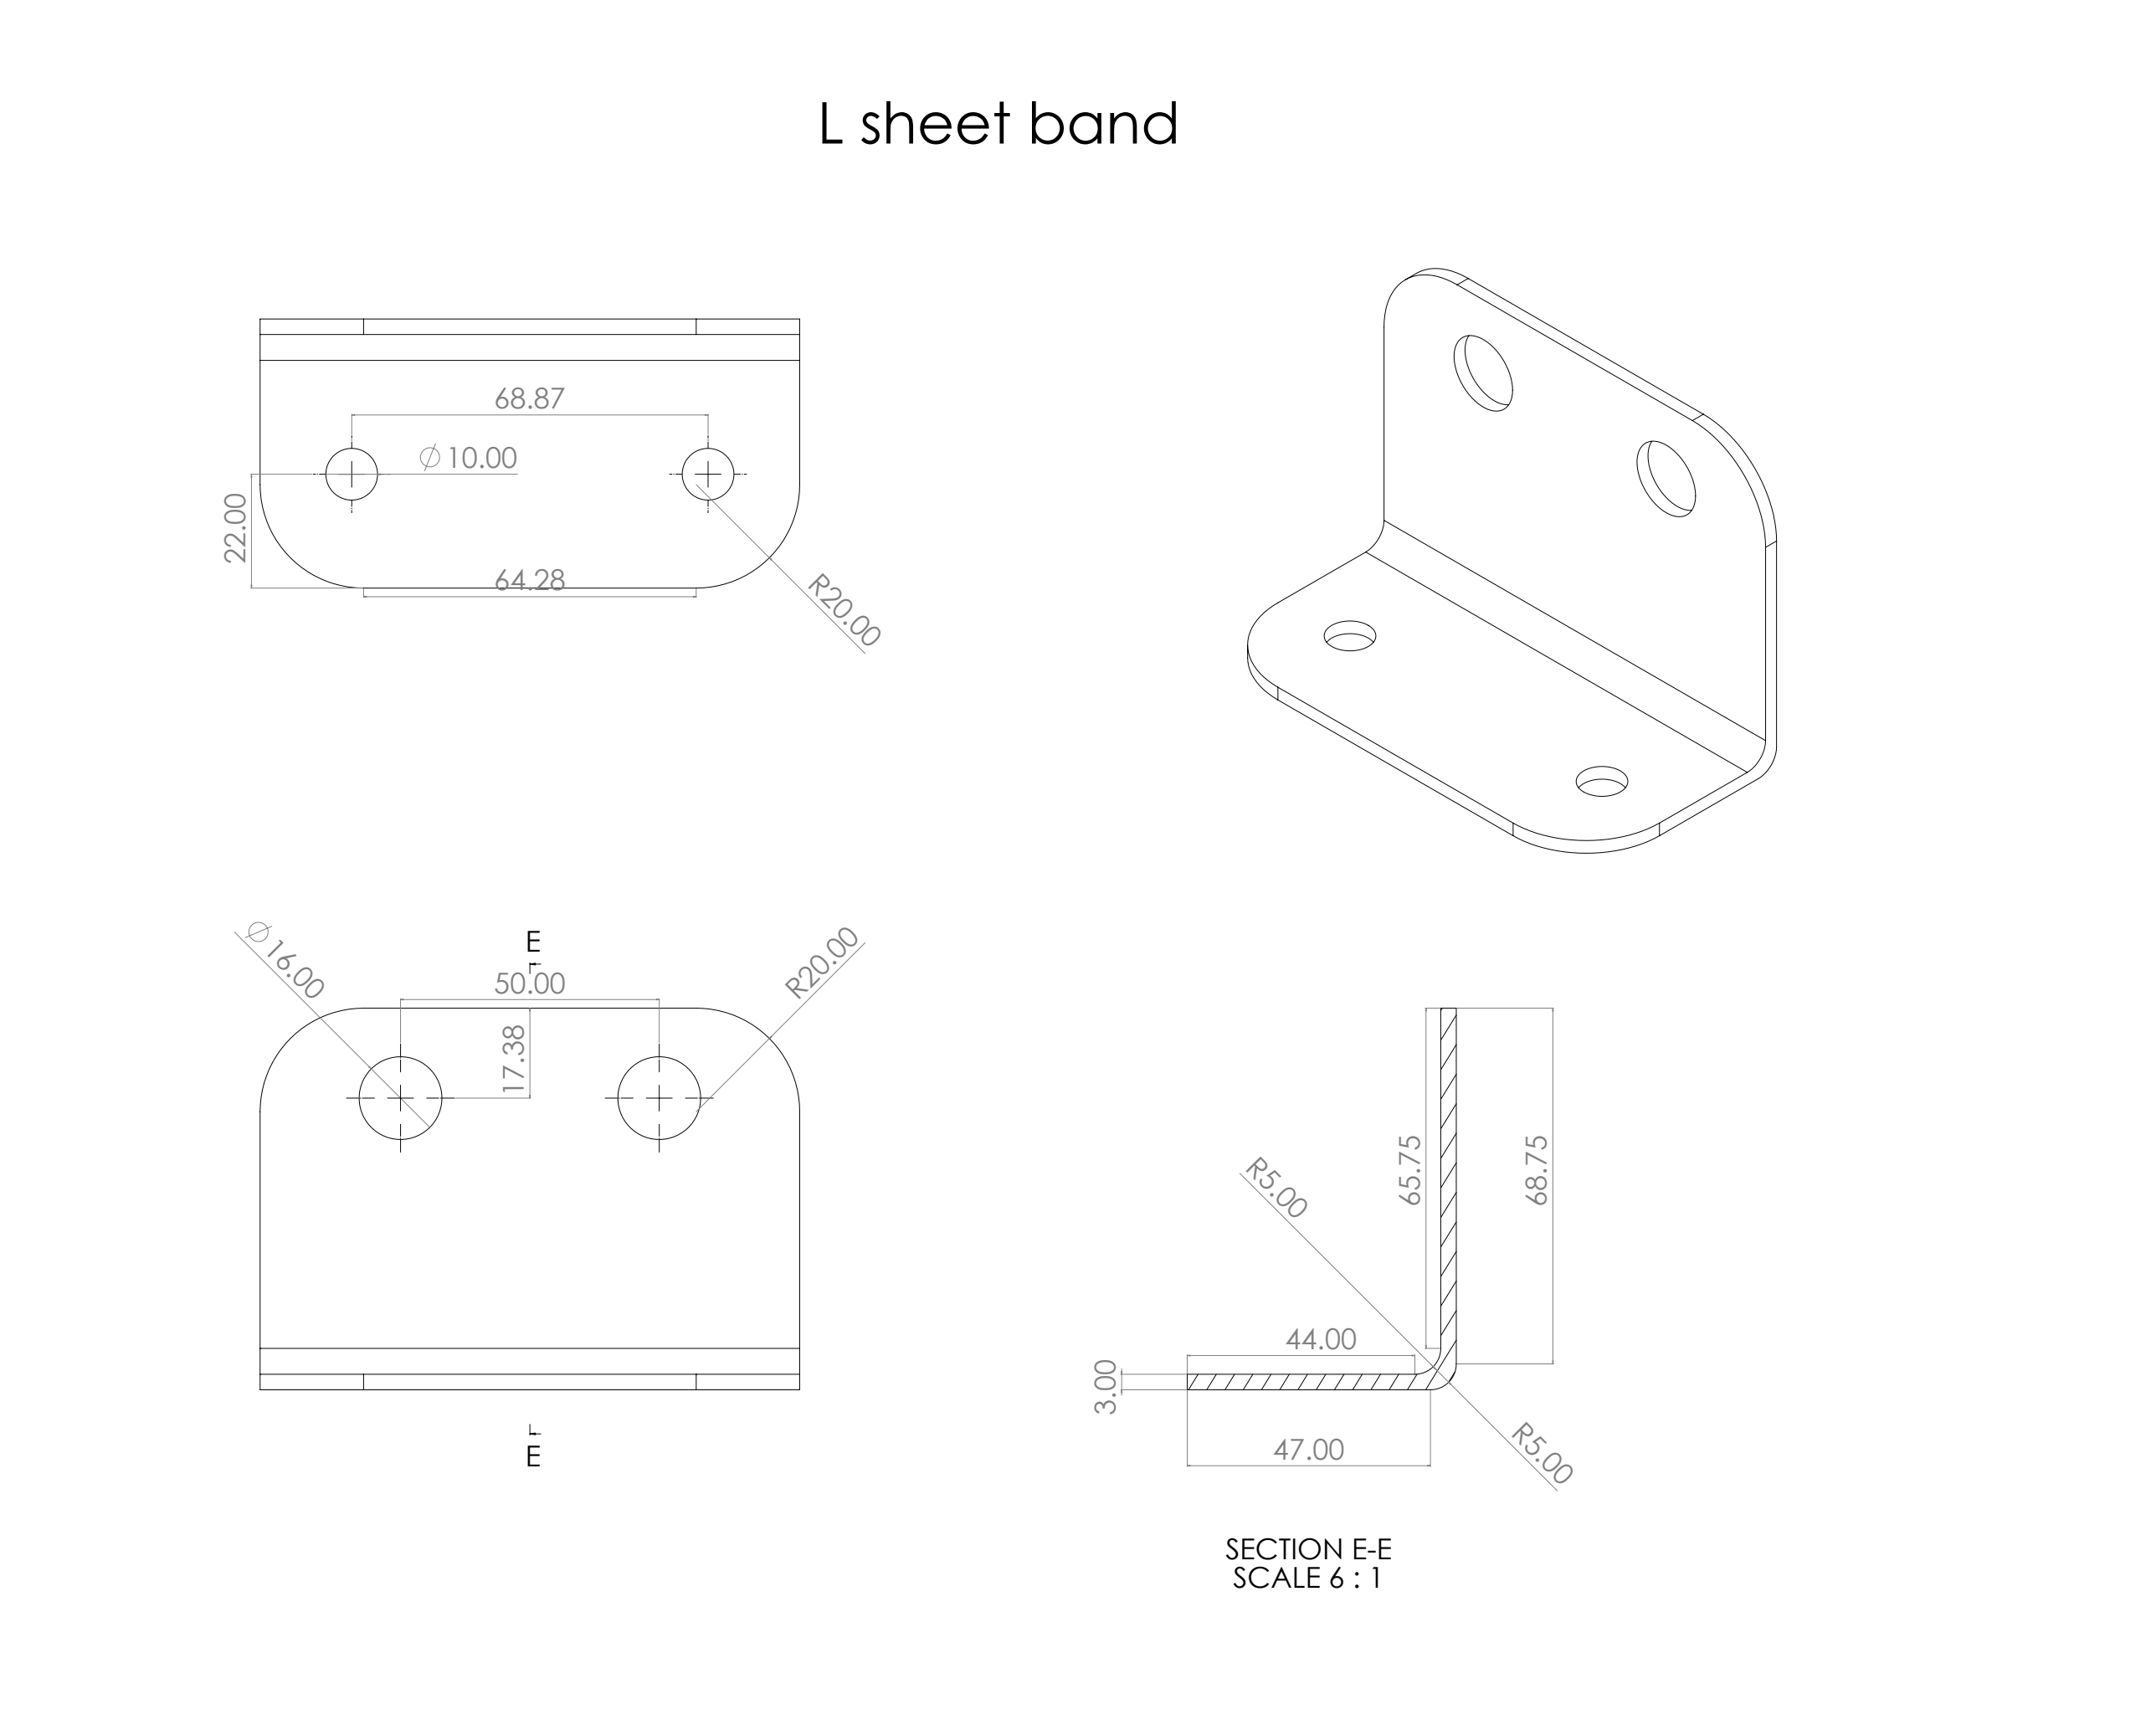
ISO-10303-21;
HEADER;
FILE_DESCRIPTION (('STEP AP214'),
    '1' );
FILE_NAME ('L sheet band.step',
    '2026-10-25T20:52:49',
    ( '' ),
    ( '' ),
    'SwSTEP 2.0',
    'SolidWorks 2025',
    '' );
FILE_SCHEMA (( 'AUTOMOTIVE_DESIGN' ));
ENDSEC;

DATA;
#211=CIRCLE ( 'NONE', #62253, 4.999999999999997335 ) ;
#499=ORIENTED_EDGE ( 'NONE', *, *, #5733, .T. ) ;
#503=CARTESIAN_POINT ( 'NONE',  ( -74.94434090351494149, -285.8906705383787994, 27.50000000000000000 ) ) ;
#530=CIRCLE ( 'NONE', #89712, 8.000000000000000000 ) ;
#590=VECTOR ( 'NONE', #42774, 1000.000000000000000 ) ;
#594=DIRECTION ( 'NONE',  ( -0.000000000000000000, 0.000000000000000000, -1.000000000000000000 ) ) ;
#669=ORIENTED_EDGE ( 'NONE', *, *, #93158, .F. ) ;
#679=EDGE_CURVE ( 'NONE', #83322, #83798, #47998, .T. ) ;
#791=EDGE_CURVE ( 'NONE', #63802, #44165, #5422, .T. ) ;
#865=ADVANCED_FACE ( 'NONE', ( #48951 ), #63665, .F. ) ;
#929=APPLICATION_CONTEXT ( 'automotive_design' ) ;
#1240=EDGE_CURVE ( 'NONE', #8882, #83322, #52548, .T. ) ;
#1428=ORIENTED_EDGE ( 'NONE', *, *, #14429, .F. ) ;
#1517=EDGE_LOOP ( 'NONE', ( #90741, #8726, #54853, #21935 ) ) ;
#1578=ORIENTED_EDGE ( 'NONE', *, *, #52624, .F. ) ;
#1600=CARTESIAN_POINT ( 'NONE',  ( 11.63197158325052172, -331.8906705383788562, 57.50000000000000000 ) ) ;
#1855=LINE ( 'NONE', #38761, #18792 ) ;
#1953=CIRCLE ( 'NONE', #71531, 5.000000000000000888 ) ;
#2043=AXIS2_PLACEMENT_3D ( 'NONE', #53323, #2683, #31562 ) ;
#2173=CIRCLE ( 'NONE', #35437, 20.00000000000000355 ) ;
#2187=VERTEX_POINT ( 'NONE', #4695 ) ;
#2252=( GEOMETRIC_REPRESENTATION_CONTEXT ( 3 ) GLOBAL_UNCERTAINTY_ASSIGNED_CONTEXT ( ( #85447 ) ) GLOBAL_UNIT_ASSIGNED_CONTEXT ( ( #20907, #28483, #57377 ) ) REPRESENTATION_CONTEXT ( 'NONE', 'WORKASPACE' ) );
#2451=VECTOR ( 'NONE', #84118, 1000.000000000000000 ) ;
#2470=CYLINDRICAL_SURFACE ( 'NONE', #63999, 5.000000000000004441 ) ;
#2536=ORIENTED_EDGE ( 'NONE', *, *, #16849, .T. ) ;
#2683=DIRECTION ( 'NONE',  ( -0.000000000000000000, 1.000000000000000000, -0.000000000000000000 ) ) ;
#2731=CARTESIAN_POINT ( 'NONE',  ( 29.33919985515026596, -285.8906705383787994, 25.50000000000000000 ) ) ;
#2748=LINE ( 'NONE', #18829, #53687 ) ;
#2764=ORIENTED_EDGE ( 'NONE', *, *, #65408, .F. ) ;
#3216=EDGE_CURVE ( 'NONE', #6956, #36970, #44399, .T. ) ;
#3291=FACE_BOUND ( 'NONE', #79678, .T. ) ;
#3472=EDGE_CURVE ( 'NONE', #2187, #79053, #42928, .T. ) ;
#3535=VECTOR ( 'NONE', #44027, 1000.000000000000000 ) ;
#3654=AXIS2_PLACEMENT_3D ( 'NONE', #5607, #71407, #86506 ) ;
#4161=DIRECTION ( 'NONE',  ( 0.000000000000000000, 0.000000000000000000, 1.000000000000000000 ) ) ;
#4211=CARTESIAN_POINT ( 'NONE',  ( 9.339199855150265961, -212.1443419142231051, 25.50000000000000000 ) ) ;
#4278=CYLINDRICAL_SURFACE ( 'NONE', #44327, 20.00000000000000355 ) ;
#4618=DIRECTION ( 'NONE',  ( -1.000000000000000000, 0.000000000000000000, 0.000000000000000000 ) ) ;
#4695=CARTESIAN_POINT ( 'NONE',  ( -57.23711263161519724, -282.8906705383787994, 47.50000000000000000 ) ) ;
#4733=ORIENTED_EDGE ( 'NONE', *, *, #61391, .F. ) ;
#4911=EDGE_CURVE ( 'NONE', #16098, #8882, #2173, .T. ) ;
#5333=ORIENTED_EDGE ( 'NONE', *, *, #71135, .T. ) ;
#5370=CARTESIAN_POINT ( 'NONE',  ( -74.94434090351494149, -232.1443419142230766, 25.50000000000000000 ) ) ;
#5378=CARTESIAN_POINT ( 'NONE',  ( -47.80257052418233599, -229.5268262511776527, 25.50000000000000000 ) ) ;
#5422=LINE ( 'NONE', #41357, #59082 ) ;
#5562=VERTEX_POINT ( 'NONE', #28040 ) ;
#5575=ORIENTED_EDGE ( 'NONE', *, *, #29965, .T. ) ;
#5605=FACE_OUTER_BOUND ( 'NONE', #91771, .T. ) ;
#5607=CARTESIAN_POINT ( 'NONE',  ( 9.339199855150265961, 0.000000000000000000, 54.50000000000000711 ) ) ;
#5696=DIRECTION ( 'NONE',  ( 0.000000000000000000, 0.000000000000000000, -1.000000000000000000 ) ) ;
#5733=EDGE_CURVE ( 'NONE', #83883, #21738, #35116, .T. ) ;
#5768=ORIENTED_EDGE ( 'NONE', *, *, #15154, .F. ) ;
#5834=CARTESIAN_POINT ( 'NONE',  ( 9.339199855150265961, -232.1443419142230766, 25.50000000000000000 ) ) ;
#5880=DIRECTION ( 'NONE',  ( -0.000000000000000000, 1.000000000000000000, -0.000000000000000000 ) ) ;
#6157=CIRCLE ( 'NONE', #21289, 5.000000000000004441 ) ;
#6190=CYLINDRICAL_SURFACE ( 'NONE', #46878, 20.00000000000000355 ) ;
#6253=ORIENTED_EDGE ( 'NONE', *, *, #81207, .T. ) ;
#6304=DIRECTION ( 'NONE',  ( 1.000000000000000000, 0.000000000000000000, -0.000000000000000000 ) ) ;
#6314=EDGE_LOOP ( 'NONE', ( #19635, #51769, #6625, #41760 ) ) ;
#6319=EDGE_LOOP ( 'NONE', ( #54530, #85626, #35666, #19153 ) ) ;
#6408=CARTESIAN_POINT ( 'NONE',  ( 11.63197158325052172, -282.8906705383787994, 52.50000000000000711 ) ) ;
#6625=ORIENTED_EDGE ( 'NONE', *, *, #39536, .F. ) ;
#6628=AXIS2_PLACEMENT_3D ( 'NONE', #41896, #20617, #63257 ) ;
#6848=EDGE_LOOP ( 'NONE', ( #78571, #68659, #63310, #44201 ) ) ;
#6956=VERTEX_POINT ( 'NONE', #81914 ) ;
#7018=CARTESIAN_POINT ( 'NONE',  ( 9.339199855150262408, -285.8906705383787994, 74.50000000000001421 ) ) ;
#7577=DIRECTION ( 'NONE',  ( 0.000000000000000000, 0.000000000000000000, 1.000000000000000000 ) ) ;
#7662=EDGE_CURVE ( 'NONE', #46169, #75426, #44596, .T. ) ;
#7944=ORIENTED_EDGE ( 'NONE', *, *, #679, .T. ) ;
#8045=AXIS2_PLACEMENT_3D ( 'NONE', #26662, #19096, #40362 ) ;
#8145=FACE_OUTER_BOUND ( 'NONE', #43480, .T. ) ;
#8181=AXIS2_PLACEMENT_3D ( 'NONE', #46720, #18327, #89815 ) ;
#8225=VERTEX_POINT ( 'NONE', #32625 ) ;
#8251=VECTOR ( 'NONE', #27083, 1000.000000000000000 ) ;
#8548=ORIENTED_EDGE ( 'NONE', *, *, #29467, .T. ) ;
#8578=DIRECTION ( 'NONE',  ( -0.000000000000000000, 1.000000000000000000, -0.000000000000000000 ) ) ;
#8726=ORIENTED_EDGE ( 'NONE', *, *, #56813, .T. ) ;
#8882=VERTEX_POINT ( 'NONE', #7018 ) ;
#9133=VERTEX_POINT ( 'NONE', #16318 ) ;
#9154=DIRECTION ( 'NONE',  ( -1.000000000000000000, 0.000000000000000000, 0.000000000000000000 ) ) ;
#9364=CIRCLE ( 'NONE', #22964, 20.00000000000000000 ) ;
#9380=ORIENTED_EDGE ( 'NONE', *, *, #53233, .F. ) ;
#9395=LINE ( 'NONE', #66263, #77580 ) ;
#9712=AXIS2_PLACEMENT_3D ( 'NONE', #80216, #9154, #87304 ) ;
#9773=CARTESIAN_POINT ( 'NONE',  ( -39.80257052418233599, -229.5268262511776527, 22.50000000000000000 ) ) ;
#9810=AXIS2_PLACEMENT_3D ( 'NONE', #43476, #35459, #57245 ) ;
#9965=ORIENTED_EDGE ( 'NONE', *, *, #36530, .F. ) ;
#9996=MECHANICAL_DESIGN_GEOMETRIC_PRESENTATION_REPRESENTATION('',(#22120),#64479);
#10069=ADVANCED_FACE ( 'NONE', ( #63173 ), #41332, .F. ) ;
#10083=ORIENTED_EDGE ( 'NONE', *, *, #3472, .F. ) ;
#10105=EDGE_CURVE ( 'NONE', #5562, #61290, #30617, .T. ) ;
#10228=DIRECTION ( 'NONE',  ( 1.000000000000000000, 0.000000000000000000, -0.000000000000000000 ) ) ;
#10503=ORIENTED_EDGE ( 'NONE', *, *, #50543, .T. ) ;
#10525=CARTESIAN_POINT ( 'NONE',  ( 9.339199855150265961, -285.8906705383787994, 54.50000000000000711 ) ) ;
#10708=DIRECTION ( 'NONE',  ( -0.000000000000000000, -1.000000000000000000, 0.000000000000000000 ) ) ;
#10810=CARTESIAN_POINT ( 'NONE',  ( 29.33919985515026596, -282.8906705383787994, 74.50000000000001421 ) ) ;
#10935=EDGE_CURVE ( 'NONE', #74457, #43263, #11136, .T. ) ;
#11136=CIRCLE ( 'NONE', #77668, 5.000000000000000888 ) ;
#11171=DIRECTION ( 'NONE',  ( -1.000000000000000000, -0.000000000000000000, 0.000000000000000000 ) ) ;
#11303=CIRCLE ( 'NONE', #85390, 8.000000000000000000 ) ;
#11310=UNCERTAINTY_MEASURE_WITH_UNIT (LENGTH_MEASURE( 1.000000000000000082E-05 ), #27421, 'distance_accuracy_value', 'NONE');
#11330=DIRECTION ( 'NONE',  ( 1.000000000000000000, 0.000000000000000000, 0.000000000000000000 ) ) ;
#11515=FACE_OUTER_BOUND ( 'NONE', #28357, .T. ) ;
#11619=DIRECTION ( 'NONE',  ( 0.000000000000000000, 0.000000000000000000, 1.000000000000000000 ) ) ;
#12027=AXIS2_PLACEMENT_3D ( 'NONE', #47486, #46093, #82550 ) ;
#12043=EDGE_LOOP ( 'NONE', ( #77514, #31253 ) ) ;
#12155=VECTOR ( 'NONE', #33086, 1000.000000000000000 ) ;
#12164=ORIENTED_EDGE ( 'NONE', *, *, #57750, .F. ) ;
#12388=EDGE_LOOP ( 'NONE', ( #84486, #669, #4733, #84122 ) ) ;
#12459=ORIENTED_EDGE ( 'NONE', *, *, #52360, .T. ) ;
#12648=ORIENTED_EDGE ( 'NONE', *, *, #28991, .T. ) ;
#12657=PRODUCT_DEFINITION_SHAPE ( 'NONE', 'NONE',  #79429 ) ;
#12775=ORIENTED_EDGE ( 'NONE', *, *, #36530, .T. ) ;
#13302=DIRECTION ( 'NONE',  ( 0.000000000000000000, 0.000000000000000000, -1.000000000000000000 ) ) ;
#13640=CARTESIAN_POINT ( 'NONE',  ( 29.33919985515026596, -285.8906705383787994, 25.50000000000000000 ) ) ;
#13872=AXIS2_PLACEMENT_3D ( 'NONE', #69873, #11171, #24921 ) ;
#14429=EDGE_CURVE ( 'NONE', #21926, #45777, #1855, .T. ) ;
#14585=CARTESIAN_POINT ( 'NONE',  ( 29.33919985515026596, -280.8906705383787994, 22.50000000000000000 ) ) ;
#14821=ORIENTED_EDGE ( 'NONE', *, *, #679, .F. ) ;
#14991=DIRECTION ( 'NONE',  ( -1.000000000000000000, 0.000000000000000000, 0.000000000000000000 ) ) ;
#15070=CIRCLE ( 'NONE', #92174, 5.000000000000004441 ) ;
#15154=EDGE_CURVE ( 'NONE', #92884, #84200, #84642, .T. ) ;
#15324=ADVANCED_FACE ( 'NONE', ( #71405, #21193, #5605 ), #36331, .F. ) ;
#15350=CARTESIAN_POINT ( 'NONE',  ( 29.33919985515026596, -277.8906705383787994, 25.50000000000000000 ) ) ;
#15367=DIRECTION ( 'NONE',  ( 0.000000000000000000, 0.000000000000000000, 1.000000000000000000 ) ) ;
#15486=FACE_OUTER_BOUND ( 'NONE', #22877, .T. ) ;
#15534=FACE_OUTER_BOUND ( 'NONE', #6848, .T. ) ;
#15602=CIRCLE ( 'NONE', #56443, 5.000000000000004441 ) ;
#15626=LINE ( 'NONE', #72924, #80151 ) ;
#15723=FACE_BOUND ( 'NONE', #92036, .T. ) ;
#15815=ORIENTED_EDGE ( 'NONE', *, *, #7662, .T. ) ;
#16098=VERTEX_POINT ( 'NONE', #52392 ) ;
#16099=DIRECTION ( 'NONE',  ( 1.000000000000000000, -0.000000000000000000, -0.000000000000000000 ) ) ;
#16318=CARTESIAN_POINT ( 'NONE',  ( -57.23711263161519724, -285.8906705383787994, 47.50000000000000000 ) ) ;
#16501=VERTEX_POINT ( 'NONE', #9773 ) ;
#16849=EDGE_CURVE ( 'NONE', #70876, #81433, #33514, .T. ) ;
#17113=DIRECTION ( 'NONE',  ( -0.000000000000000000, 1.000000000000000000, -0.000000000000000000 ) ) ;
#17170=CIRCLE ( 'NONE', #86710, 8.000000000000000000 ) ;
#17251=ORIENTED_EDGE ( 'NONE', *, *, #57750, .T. ) ;
#17403=CARTESIAN_POINT ( 'NONE',  ( 11.63197158325052172, -285.8906705383787994, 52.50000000000000711 ) ) ;
#17496=ORIENTED_EDGE ( 'NONE', *, *, #32434, .T. ) ;
#17684=DIRECTION ( 'NONE',  ( -0.000000000000000000, 1.000000000000000000, -0.000000000000000000 ) ) ;
#17831=CARTESIAN_POINT ( 'NONE',  ( -54.94434090351493438, -285.8906705383787994, 54.50000000000000711 ) ) ;
#17868=DIRECTION ( 'NONE',  ( 0.000000000000000000, 1.000000000000000000, -0.000000000000000000 ) ) ;
#17920=CARTESIAN_POINT ( 'NONE',  ( -54.94434090351493438, -232.1443419142230766, 25.50000000000000000 ) ) ;
#18327=DIRECTION ( 'NONE',  ( -0.000000000000000000, -0.000000000000000000, -1.000000000000000000 ) ) ;
#18328=DIRECTION ( 'NONE',  ( -0.000000000000000000, -0.000000000000000000, -1.000000000000000000 ) ) ;
#18792=VECTOR ( 'NONE', #53442, 1000.000000000000000 ) ;
#18797=CARTESIAN_POINT ( 'NONE',  ( 29.33919985515026596, -232.1443419142230766, 25.50000000000000000 ) ) ;
#18813=ORIENTED_EDGE ( 'NONE', *, *, #92502, .T. ) ;
#18829=CARTESIAN_POINT ( 'NONE',  ( -74.94434090351494149, -285.8906705383787994, 25.50000000000000000 ) ) ;
#18940=AXIS2_PLACEMENT_3D ( 'NONE', #90959, #40773, #33703 ) ;
#19096=DIRECTION ( 'NONE',  ( 0.000000000000000000, 0.000000000000000000, 1.000000000000000000 ) ) ;
#19153=ORIENTED_EDGE ( 'NONE', *, *, #23961, .F. ) ;
#19228=CARTESIAN_POINT ( 'NONE',  ( -54.94434090351493438, 0.000000000000000000, 74.50000000000001421 ) ) ;
#19629=EDGE_LOOP ( 'NONE', ( #76225, #76329, #50740, #51309, #86118, #58445, #72981, #2536 ) ) ;
#19635=ORIENTED_EDGE ( 'NONE', *, *, #4911, .F. ) ;
#20025=DIRECTION ( 'NONE',  ( -1.000000000000000000, 0.000000000000000000, 0.000000000000000000 ) ) ;
#20206=DIRECTION ( 'NONE',  ( -0.000000000000000000, 1.000000000000000000, -0.000000000000000000 ) ) ;
#20284=APPLICATION_CONTEXT ( 'automotive_design' ) ;
#20504=DIRECTION ( 'NONE',  ( 0.000000000000000000, 0.000000000000000000, -1.000000000000000000 ) ) ;
#20549=DIRECTION ( 'NONE',  ( 0.000000000000000000, 0.000000000000000000, -1.000000000000000000 ) ) ;
#20606=CARTESIAN_POINT ( 'NONE',  ( 2.197429475817664013, -229.5268262511776527, 25.50000000000000000 ) ) ;
#20617=DIRECTION ( 'NONE',  ( 0.000000000000000000, -1.000000000000000000, 0.000000000000000000 ) ) ;
#20640=DIRECTION ( 'NONE',  ( 0.000000000000000000, 0.000000000000000000, 1.000000000000000000 ) ) ;
#20772=ORIENTED_EDGE ( 'NONE', *, *, #92502, .F. ) ;
#20857=CARTESIAN_POINT ( 'NONE',  ( 0.000000000000000000, 0.000000000000000000, 74.50000000000001421 ) ) ;
#20907=( LENGTH_UNIT ( ) NAMED_UNIT ( * ) SI_UNIT ( .MILLI., .METRE. ) );
#21095=EDGE_CURVE ( 'NONE', #75426, #34536, #47579, .T. ) ;
#21193=FACE_BOUND ( 'NONE', #77112, .T. ) ;
#21225=AXIS2_PLACEMENT_3D ( 'NONE', #20857, #86171, #58263 ) ;
#21249=DIRECTION ( 'NONE',  ( -1.000000000000000000, 0.000000000000000000, 0.000000000000000000 ) ) ;
#21289=AXIS2_PLACEMENT_3D ( 'NONE', #70282, #49419, #20549 ) ;
#21365=ORIENTED_EDGE ( 'NONE', *, *, #29965, .F. ) ;
#21433=DIRECTION ( 'NONE',  ( 0.000000000000000000, 0.000000000000000000, -1.000000000000000000 ) ) ;
#21630=CARTESIAN_POINT ( 'NONE',  ( 9.339199855150265961, -232.1443419142230766, 22.50000000000000000 ) ) ;
#21738=VERTEX_POINT ( 'NONE', #80210 ) ;
#21756=EDGE_CURVE ( 'NONE', #93354, #36970, #78821, .T. ) ;
#21926=VERTEX_POINT ( 'NONE', #15350 ) ;
#21935=ORIENTED_EDGE ( 'NONE', *, *, #28991, .F. ) ;
#22120=STYLED_ITEM('',(#93766),#91539);
#22181=CARTESIAN_POINT ( 'NONE',  ( -47.80257052418233599, -229.5268262511776527, 25.50000000000000000 ) ) ;
#22216=LINE ( 'NONE', #58223, #67039 ) ;
#22241=CARTESIAN_POINT ( 'NONE',  ( -57.23711263161519724, -285.8906705383787994, 52.50000000000000711 ) ) ;
#22448=EDGE_CURVE ( 'NONE', #63080, #8882, #74495, .T. ) ;
#22580=EDGE_CURVE ( 'NONE', #46169, #33107, #59378, .T. ) ;
#22877=EDGE_LOOP ( 'NONE', ( #47031, #76243, #24143, #36824 ) ) ;
#22964=AXIS2_PLACEMENT_3D ( 'NONE', #21630, #41986, #14991 ) ;
#22975=VECTOR ( 'NONE', #82780, 1000.000000000000000 ) ;
#23071=CARTESIAN_POINT ( 'NONE',  ( -54.94434090351493438, -282.8906705383787994, 74.50000000000001421 ) ) ;
#23097=AXIS2_PLACEMENT_3D ( 'NONE', #90759, #4161, #4618 ) ;
#23178=DIRECTION ( 'NONE',  ( 0.000000000000000000, 1.000000000000000000, -0.000000000000000000 ) ) ;
#23659=ADVANCED_FACE ( 'NONE', ( #25815 ), #40464, .F. ) ;
#23961=EDGE_CURVE ( 'NONE', #81433, #74457, #24900, .T. ) ;
#24143=ORIENTED_EDGE ( 'NONE', *, *, #22580, .T. ) ;
#24169=EDGE_LOOP ( 'NONE', ( #6253, #499, #39864, #87621 ) ) ;
#24492=CARTESIAN_POINT ( 'NONE',  ( 29.33919985515026596, -277.8906705383787994, 30.50000000000000000 ) ) ;
#24517=AXIS2_PLACEMENT_3D ( 'NONE', #17831, #10708, #39564 ) ;
#24668=CIRCLE ( 'NONE', #8045, 8.000000000000000000 ) ;
#24768=CARTESIAN_POINT ( 'NONE',  ( -54.94434090351493438, -285.8906705383787994, 74.50000000000001421 ) ) ;
#24900=LINE ( 'NONE', #53780, #92639 ) ;
#24921=DIRECTION ( 'NONE',  ( 0.000000000000000000, 0.000000000000000000, -1.000000000000000000 ) ) ;
#24967=DIRECTION ( 'NONE',  ( 0.000000000000000000, 1.000000000000000000, -0.000000000000000000 ) ) ;
#25368=DIRECTION ( 'NONE',  ( 1.000000000000000000, -0.000000000000000000, -0.000000000000000000 ) ) ;
#25784=EDGE_CURVE ( 'NONE', #9133, #74935, #15602, .T. ) ;
#25792=ORIENTED_EDGE ( 'NONE', *, *, #50543, .F. ) ;
#25815=FACE_OUTER_BOUND ( 'NONE', #49889, .T. ) ;
#25886=DIRECTION ( 'NONE',  ( 0.000000000000000000, 0.000000000000000000, 1.000000000000000000 ) ) ;
#25996=AXIS2_PLACEMENT_3D ( 'NONE', #60677, #17113, #33180 ) ;
#26044=CARTESIAN_POINT ( 'NONE',  ( -54.94434090351493438, -232.1443419142230766, 25.50000000000000000 ) ) ;
#26074=DIRECTION ( 'NONE',  ( -0.000000000000000000, -1.000000000000000000, -0.000000000000000000 ) ) ;
#26154=VECTOR ( 'NONE', #20504, 1000.000000000000000 ) ;
#26205=ORIENTED_EDGE ( 'NONE', *, *, #22448, .F. ) ;
#26238=CARTESIAN_POINT ( 'NONE',  ( -74.94434090351494149, -282.8906705383787994, 74.50000000000001421 ) ) ;
#26379=ORIENTED_EDGE ( 'NONE', *, *, #23961, .T. ) ;
#26662=CARTESIAN_POINT ( 'NONE',  ( 2.197429475817664013, -229.5268262511776527, 22.50000000000000000 ) ) ;
#26667=CARTESIAN_POINT ( 'NONE',  ( 29.33919985515026596, -285.8906705383787994, 27.50000000000000000 ) ) ;
#26772=DIRECTION ( 'NONE',  ( -1.000000000000000000, 0.000000000000000000, 0.000000000000000000 ) ) ;
#26785=CARTESIAN_POINT ( 'NONE',  ( 29.33919985515026596, -280.8906705383787994, 27.50000000000000000 ) ) ;
#26852=ORIENTED_EDGE ( 'NONE', *, *, #10935, .T. ) ;
#27083=DIRECTION ( 'NONE',  ( -0.000000000000000000, -0.000000000000000000, -1.000000000000000000 ) ) ;
#27156=CARTESIAN_POINT ( 'NONE',  ( 2.197429475817664013, -229.5268262511776527, 25.50000000000000000 ) ) ;
#27209=ORIENTED_EDGE ( 'NONE', *, *, #52624, .T. ) ;
#27373=CARTESIAN_POINT ( 'NONE',  ( -74.94434090351494149, -282.8906705383787994, 54.50000000000000711 ) ) ;
#27421=( LENGTH_UNIT ( ) NAMED_UNIT ( * ) SI_UNIT ( .MILLI., .METRE. ) );
#27422=DIRECTION ( 'NONE',  ( -0.000000000000000000, 0.000000000000000000, -1.000000000000000000 ) ) ;
#27491=PLANE ( 'NONE',  #21225 ) ;
#28040=CARTESIAN_POINT ( 'NONE',  ( -5.802570524182335987, -229.5268262511776527, 25.50000000000000000 ) ) ;
#28085=PRODUCT_DEFINITION_FORMATION_WITH_SPECIFIED_SOURCE ( 'ANY', '', #64119, .NOT_KNOWN. ) ;
#28273=EDGE_CURVE ( 'NONE', #36049, #77270, #1953, .T. ) ;
#28357=EDGE_LOOP ( 'NONE', ( #14821, #80378, #88183, #27209, #86593, #61328 ) ) ;
#28483=( NAMED_UNIT ( * ) PLANE_ANGLE_UNIT ( ) SI_UNIT ( $, .RADIAN. ) );
#28635=DIRECTION ( 'NONE',  ( -1.000000000000000000, 0.000000000000000000, 0.000000000000000000 ) ) ;
#28872=AXIS2_PLACEMENT_3D ( 'NONE', #70738, #34280, #91055 ) ;
#28991=EDGE_CURVE ( 'NONE', #74935, #79053, #81498, .T. ) ;
#29086=ORIENTED_EDGE ( 'NONE', *, *, #53233, .T. ) ;
#29302=AXIS2_PLACEMENT_3D ( 'NONE', #44842, #73745, #37735 ) ;
#29467=EDGE_CURVE ( 'NONE', #92884, #16098, #90908, .T. ) ;
#29563=ORIENTED_EDGE ( 'NONE', *, *, #14429, .T. ) ;
#29758=CYLINDRICAL_SURFACE ( 'NONE', #81041, 8.000000000000000000 ) ;
#29881=EDGE_CURVE ( 'NONE', #6956, #70876, #40114, .T. ) ;
#29965=EDGE_CURVE ( 'NONE', #45777, #90307, #63972, .T. ) ;
#30027=CARTESIAN_POINT ( 'NONE',  ( 29.33919985515026596, -212.1443419142231051, 22.50000000000000000 ) ) ;
#30300=ORIENTED_EDGE ( 'NONE', *, *, #80845, .T. ) ;
#30373=ORIENTED_EDGE ( 'NONE', *, *, #47352, .F. ) ;
#30617=LINE ( 'NONE', #53315, #48856 ) ;
#30653=CARTESIAN_POINT ( 'NONE',  ( 10.19742947581766401, -229.5268262511776527, 25.50000000000000000 ) ) ;
#30672=AXIS2_PLACEMENT_3D ( 'NONE', #83569, #26772, #11619 ) ;
#30676=DIRECTION ( 'NONE',  ( -1.000000000000000000, 0.000000000000000000, 0.000000000000000000 ) ) ;
#30839=EDGE_CURVE ( 'NONE', #93354, #8225, #9364, .T. ) ;
#31105=PLANE ( 'NONE',  #42859 ) ;
#31207=CARTESIAN_POINT ( 'NONE',  ( -74.94434090351494149, -280.8906705383787994, 22.50000000000000000 ) ) ;
#31253=ORIENTED_EDGE ( 'NONE', *, *, #87350, .F. ) ;
#31343=VERTEX_POINT ( 'NONE', #66581 ) ;
#31562=DIRECTION ( 'NONE',  ( 0.000000000000000000, 0.000000000000000000, 1.000000000000000000 ) ) ;
#31628=DIRECTION ( 'NONE',  ( -0.000000000000000000, -0.000000000000000000, -1.000000000000000000 ) ) ;
#32103=EDGE_CURVE ( 'NONE', #63802, #31343, #80773, .T. ) ;
#32371=CYLINDRICAL_SURFACE ( 'NONE', #12027, 5.000000000000000888 ) ;
#32426=ORIENTED_EDGE ( 'NONE', *, *, #1240, .T. ) ;
#32434=EDGE_CURVE ( 'NONE', #43263, #8225, #79181, .T. ) ;
#32625=CARTESIAN_POINT ( 'NONE',  ( 29.33919985515026596, -232.1443419142230766, 22.50000000000000000 ) ) ;
#33001=CARTESIAN_POINT ( 'NONE',  ( -57.23711263161519724, -282.8906705383787994, 52.50000000000000711 ) ) ;
#33006=ORIENTED_EDGE ( 'NONE', *, *, #35340, .T. ) ;
#33032=CARTESIAN_POINT ( 'NONE',  ( -74.94434090351494149, -212.1443419142231051, 22.50000000000000000 ) ) ;
#33086=DIRECTION ( 'NONE',  ( 0.000000000000000000, 0.000000000000000000, -1.000000000000000000 ) ) ;
#33107=VERTEX_POINT ( 'NONE', #62047 ) ;
#33180=DIRECTION ( 'NONE',  ( 1.040834085586084059E-15, 0.000000000000000000, -1.000000000000000000 ) ) ;
#33313=ORIENTED_EDGE ( 'NONE', *, *, #71135, .F. ) ;
#33367=EDGE_LOOP ( 'NONE', ( #21365, #84423, #72576, #9380 ) ) ;
#33514=CIRCLE ( 'NONE', #13872, 5.000000000000000888 ) ;
#33634=ADVANCED_FACE ( 'NONE', ( #85220 ), #4278, .T. ) ;
#33703=DIRECTION ( 'NONE',  ( 1.000000000000000000, 0.000000000000000000, 0.000000000000000000 ) ) ;
#33753=AXIS2_PLACEMENT_3D ( 'NONE', #35074, #57802, #78642 ) ;
#34014=FACE_OUTER_BOUND ( 'NONE', #6314, .T. ) ;
#34048=DIRECTION ( 'NONE',  ( -0.000000000000000000, 1.000000000000000000, -0.000000000000000000 ) ) ;
#34055=ORIENTED_EDGE ( 'NONE', *, *, #92271, .F. ) ;
#34063=FACE_OUTER_BOUND ( 'NONE', #64380, .T. ) ;
#34208=ORIENTED_EDGE ( 'NONE', *, *, #30839, .T. ) ;
#34280=DIRECTION ( 'NONE',  ( 0.000000000000000000, 1.000000000000000000, 0.000000000000000000 ) ) ;
#34287=DIRECTION ( 'NONE',  ( -0.000000000000000000, -0.000000000000000000, -1.000000000000000000 ) ) ;
#34338=CYLINDRICAL_SURFACE ( 'NONE', #74747, 8.000000000000000000 ) ;
#34352=CARTESIAN_POINT ( 'NONE',  ( 2.197429475817664013, -229.5268262511776527, 22.50000000000000000 ) ) ;
#34536=VERTEX_POINT ( 'NONE', #54327 ) ;
#34589=CARTESIAN_POINT ( 'NONE',  ( -47.80257052418233599, -229.5268262511776527, 22.50000000000000000 ) ) ;
#35074=CARTESIAN_POINT ( 'NONE',  ( 2.197429475817664013, -229.5268262511776527, 25.50000000000000000 ) ) ;
#35116=LINE ( 'NONE', #91928, #8251 ) ;
#35139=CARTESIAN_POINT ( 'NONE',  ( -47.80257052418233599, -229.5268262511776527, 25.50000000000000000 ) ) ;
#35167=CYLINDRICAL_SURFACE ( 'NONE', #47135, 20.00000000000000000 ) ;
#35281=AXIS2_PLACEMENT_3D ( 'NONE', #27156, #48927, #38643 ) ;
#35319=EDGE_CURVE ( 'NONE', #52696, #6956, #55551, .T. ) ;
#35340=EDGE_CURVE ( 'NONE', #21738, #61290, #24668, .T. ) ;
#35341=ADVANCED_FACE ( 'NONE', ( #92436, #76391, #11515 ), #41784, .F. ) ;
#35437=AXIS2_PLACEMENT_3D ( 'NONE', #10525, #54549, #82507 ) ;
#35459=DIRECTION ( 'NONE',  ( 0.000000000000000000, 0.000000000000000000, 1.000000000000000000 ) ) ;
#35584=AXIS2_PLACEMENT_3D ( 'NONE', #35926, #27422, #21249 ) ;
#35614=ORIENTED_EDGE ( 'NONE', *, *, #4911, .T. ) ;
#35649=FACE_OUTER_BOUND ( 'NONE', #79480, .T. ) ;
#35666=ORIENTED_EDGE ( 'NONE', *, *, #10935, .F. ) ;
#35899=ORIENTED_EDGE ( 'NONE', *, *, #28273, .F. ) ;
#35926=CARTESIAN_POINT ( 'NONE',  ( 0.000000000000000000, 0.000000000000000000, 22.50000000000000000 ) ) ;
#36049=VERTEX_POINT ( 'NONE', #57882 ) ;
#36093=CIRCLE ( 'NONE', #37563, 4.999999999999997335 ) ;
#36198=FACE_OUTER_BOUND ( 'NONE', #40803, .T. ) ;
#36228=CARTESIAN_POINT ( 'NONE',  ( -74.94434090351494149, -277.8906705383787994, 25.50000000000000000 ) ) ;
#36331=PLANE ( 'NONE',  #80424 ) ;
#36472=DIRECTION ( 'NONE',  ( -0.000000000000000000, -0.000000000000000000, -1.000000000000000000 ) ) ;
#36530=EDGE_CURVE ( 'NONE', #16501, #44165, #17170, .T. ) ;
#36561=DIRECTION ( 'NONE',  ( -1.000000000000000000, 0.000000000000000000, 0.000000000000000000 ) ) ;
#36824=ORIENTED_EDGE ( 'NONE', *, *, #47352, .T. ) ;
#36970=VERTEX_POINT ( 'NONE', #48301 ) ;
#37356=DIRECTION ( 'NONE',  ( -1.000000000000000000, 0.000000000000000000, 0.000000000000000000 ) ) ;
#37563=AXIS2_PLACEMENT_3D ( 'NONE', #6408, #72216, #15367 ) ;
#37735=DIRECTION ( 'NONE',  ( 0.000000000000000000, 0.000000000000000000, 1.000000000000000000 ) ) ;
#37947=VECTOR ( 'NONE', #34048, 1000.000000000000000 ) ;
#38319=CARTESIAN_POINT ( 'NONE',  ( -74.94434090351494149, -282.8906705383787994, 74.50000000000001421 ) ) ;
#38357=VECTOR ( 'NONE', #58106, 1000.000000000000000 ) ;
#38442=CIRCLE ( 'NONE', #47501, 20.00000000000000355 ) ;
#38643=DIRECTION ( 'NONE',  ( -1.000000000000000000, 0.000000000000000000, 0.000000000000000000 ) ) ;
#38761=CARTESIAN_POINT ( 'NONE',  ( 29.33919985515026596, -212.1443419142231051, 25.50000000000000000 ) ) ;
#39129=ADVANCED_FACE ( 'NONE', ( #34014 ), #91752, .T. ) ;
#39152=ORIENTED_EDGE ( 'NONE', *, *, #65408, .T. ) ;
#39326=DIRECTION ( 'NONE',  ( -0.000000000000000000, 1.000000000000000000, -0.000000000000000000 ) ) ;
#39536=EDGE_CURVE ( 'NONE', #83322, #92884, #38442, .T. ) ;
#39564=DIRECTION ( 'NONE',  ( 0.000000000000000000, 0.000000000000000000, 1.000000000000000000 ) ) ;
#39699=VECTOR ( 'NONE', #26074, 1000.000000000000000 ) ;
#39706=VERTEX_POINT ( 'NONE', #27373 ) ;
#39713=ORIENTED_EDGE ( 'NONE', *, *, #5733, .F. ) ;
#39753=EDGE_LOOP ( 'NONE', ( #30373, #64019 ) ) ;
#39864=ORIENTED_EDGE ( 'NONE', *, *, #72960, .F. ) ;
#39878=ADVANCED_FACE ( 'NONE', ( #15486 ), #52395, .F. ) ;
#39909=VERTEX_POINT ( 'NONE', #88376 ) ;
#40088=ADVANCED_FACE ( 'NONE', ( #66165 ), #31105, .F. ) ;
#40114=LINE ( 'NONE', #33032, #85084 ) ;
#40362=DIRECTION ( 'NONE',  ( 1.000000000000000000, 0.000000000000000000, 0.000000000000000000 ) ) ;
#40464=PLANE ( 'NONE',  #30672 ) ;
#40773=DIRECTION ( 'NONE',  ( 0.000000000000000000, 0.000000000000000000, 1.000000000000000000 ) ) ;
#40803=EDGE_LOOP ( 'NONE', ( #39713, #46805, #79734, #85419 ) ) ;
#41332=CYLINDRICAL_SURFACE ( 'NONE', #35281, 8.000000000000000000 ) ;
#41357=CARTESIAN_POINT ( 'NONE',  ( -55.80257052418233599, -229.5268262511776527, 25.50000000000000000 ) ) ;
#41575=CLOSED_SHELL ( 'NONE', ( #865, #79292, #91837, #10069, #59068, #88356, #23659, #72985, #40088, #15324, #68204, #58558, #35341, #76716, #74313, #69031, #83824, #39878, #39129, #76387, #33634, #58733 ) ) ;
#41722=EDGE_LOOP ( 'NONE', ( #88032, #39152, #78459, #29086 ) ) ;
#41760=ORIENTED_EDGE ( 'NONE', *, *, #1240, .F. ) ;
#41784=PLANE ( 'NONE',  #60990 ) ;
#41790=CARTESIAN_POINT ( 'NONE',  ( -57.23711263161519724, -285.8906705383787994, 57.50000000000000711 ) ) ;
#41896=CARTESIAN_POINT ( 'NONE',  ( 29.33919985515026596, -212.1443419142231051, 25.50000000000000000 ) ) ;
#41986=DIRECTION ( 'NONE',  ( -0.000000000000000000, -0.000000000000000000, -1.000000000000000000 ) ) ;
#41988=ORIENTED_EDGE ( 'NONE', *, *, #32434, .F. ) ;
#42152=AXIS2_PLACEMENT_3D ( 'NONE', #86276, #43662, #72557 ) ;
#42296=VECTOR ( 'NONE', #36472, 1000.000000000000000 ) ;
#42631=AXIS2_PLACEMENT_3D ( 'NONE', #5378, #92445, #20025 ) ;
#42774=DIRECTION ( 'NONE',  ( -1.000000000000000000, -0.000000000000000000, -0.000000000000000000 ) ) ;
#42829=DIRECTION ( 'NONE',  ( -1.000000000000000000, 0.000000000000000000, 0.000000000000000000 ) ) ;
#42859=AXIS2_PLACEMENT_3D ( 'NONE', #81732, #10228, #89289 ) ;
#42928=CIRCLE ( 'NONE', #86779, 5.000000000000004441 ) ;
#43228=FACE_OUTER_BOUND ( 'NONE', #1517, .T. ) ;
#43263=VERTEX_POINT ( 'NONE', #14585 ) ;
#43476=CARTESIAN_POINT ( 'NONE',  ( 2.197429475817664013, -229.5268262511776527, 25.50000000000000000 ) ) ;
#43480=EDGE_LOOP ( 'NONE', ( #69013, #5333, #30300, #12459, #29563, #5575 ) ) ;
#43662=DIRECTION ( 'NONE',  ( 0.000000000000000000, 0.000000000000000000, 1.000000000000000000 ) ) ;
#44027=DIRECTION ( 'NONE',  ( 0.000000000000000000, -1.000000000000000000, 0.000000000000000000 ) ) ;
#44165=VERTEX_POINT ( 'NONE', #71298 ) ;
#44201=ORIENTED_EDGE ( 'NONE', *, *, #791, .F. ) ;
#44327=AXIS2_PLACEMENT_3D ( 'NONE', #26044, #5696, #54929 ) ;
#44399=CIRCLE ( 'NONE', #8181, 20.00000000000000355 ) ;
#44596=CIRCLE ( 'NONE', #80833, 4.999999999999997335 ) ;
#44842=CARTESIAN_POINT ( 'NONE',  ( -57.23711263161519724, -331.8906705383788562, 52.50000000000000711 ) ) ;
#44863=( NAMED_UNIT ( * ) PLANE_ANGLE_UNIT ( ) SI_UNIT ( $, .RADIAN. ) );
#45243=VECTOR ( 'NONE', #47625, 1000.000000000000000 ) ;
#45293=ORIENTED_EDGE ( 'NONE', *, *, #35319, .F. ) ;
#45408=CARTESIAN_POINT ( 'NONE',  ( -74.94434090351494149, -282.8906705383787994, 30.50000000000000000 ) ) ;
#45513=CARTESIAN_POINT ( 'NONE',  ( -57.23711263161519724, -331.8906705383788562, 52.50000000000000711 ) ) ;
#45777=VERTEX_POINT ( 'NONE', #80972 ) ;
#45888=CARTESIAN_POINT ( 'NONE',  ( -74.94434090351494149, -232.1443419142230766, 25.50000000000000000 ) ) ;
#45909=CARTESIAN_POINT ( 'NONE',  ( 9.339199855150265961, 0.000000000000000000, 74.50000000000001421 ) ) ;
#45958=VECTOR ( 'NONE', #8578, 1000.000000000000000 ) ;
#46093=DIRECTION ( 'NONE',  ( 1.000000000000000000, 0.000000000000000000, 0.000000000000000000 ) ) ;
#46169=VERTEX_POINT ( 'NONE', #88052 ) ;
#46720=CARTESIAN_POINT ( 'NONE',  ( -54.94434090351493438, -232.1443419142230766, 22.50000000000000000 ) ) ;
#46805=ORIENTED_EDGE ( 'NONE', *, *, #87350, .T. ) ;
#46878=AXIS2_PLACEMENT_3D ( 'NONE', #79096, #78625, #13302 ) ;
#47031=ORIENTED_EDGE ( 'NONE', *, *, #21095, .F. ) ;
#47135=AXIS2_PLACEMENT_3D ( 'NONE', #5834, #56506, #85364 ) ;
#47206=VECTOR ( 'NONE', #17684, 1000.000000000000000 ) ;
#47352=EDGE_CURVE ( 'NONE', #33107, #34536, #36093, .T. ) ;
#47486=CARTESIAN_POINT ( 'NONE',  ( -74.94434090351494149, -277.8906705383787994, 30.50000000000000000 ) ) ;
#47501=AXIS2_PLACEMENT_3D ( 'NONE', #58135, #85123, #86046 ) ;
#47507=ORIENTED_EDGE ( 'NONE', *, *, #29881, .F. ) ;
#47579=LINE ( 'NONE', #56599, #79010 ) ;
#47625=DIRECTION ( 'NONE',  ( 0.000000000000000000, -1.000000000000000000, 0.000000000000000000 ) ) ;
#47642=CARTESIAN_POINT ( 'NONE',  ( 29.33919985515026596, -282.8906705383787994, 30.50000000000000000 ) ) ;
#47953=FACE_OUTER_BOUND ( 'NONE', #54918, .T. ) ;
#47998=LINE ( 'NONE', #26238, #590 ) ;
#48225=LINE ( 'NONE', #77127, #37947 ) ;
#48301=CARTESIAN_POINT ( 'NONE',  ( -54.94434090351493438, -212.1443419142231051, 22.50000000000000000 ) ) ;
#48682=ORIENTED_EDGE ( 'NONE', *, *, #55414, .T. ) ;
#48747=ORIENTED_EDGE ( 'NONE', *, *, #52360, .F. ) ;
#48856=VECTOR ( 'NONE', #87426, 1000.000000000000000 ) ;
#48927=DIRECTION ( 'NONE',  ( -0.000000000000000000, -0.000000000000000000, -1.000000000000000000 ) ) ;
#48951=FACE_OUTER_BOUND ( 'NONE', #83487, .T. ) ;
#49044=CARTESIAN_POINT ( 'NONE',  ( -57.23711263161519724, -285.8906705383787994, 52.50000000000000711 ) ) ;
#49364=EDGE_CURVE ( 'NONE', #44165, #16501, #82979, .T. ) ;
#49419=DIRECTION ( 'NONE',  ( 0.000000000000000000, 1.000000000000000000, -0.000000000000000000 ) ) ;
#49439=VERTEX_POINT ( 'NONE', #58819 ) ;
#49651=EDGE_LOOP ( 'NONE', ( #54403, #12775 ) ) ;
#49889=EDGE_LOOP ( 'NONE', ( #5768, #8548, #72077, #26852, #17496, #82008, #1428, #18813 ) ) ;
#50118=FACE_BOUND ( 'NONE', #49651, .T. ) ;
#50265=EDGE_CURVE ( 'NONE', #83798, #63080, #70378, .T. ) ;
#50515=LINE ( 'NONE', #79413, #38357 ) ;
#50543=EDGE_CURVE ( 'NONE', #74935, #9133, #15070, .T. ) ;
#50740=ORIENTED_EDGE ( 'NONE', *, *, #52524, .T. ) ;
#50785=CARTESIAN_POINT ( 'NONE',  ( -74.94434090351494149, -277.8906705383787994, 30.50000000000000000 ) ) ;
#51241=ORIENTED_EDGE ( 'NONE', *, *, #56813, .F. ) ;
#51309=ORIENTED_EDGE ( 'NONE', *, *, #28273, .T. ) ;
#51591=LINE ( 'NONE', #45408, #54387 ) ;
#51769=ORIENTED_EDGE ( 'NONE', *, *, #29467, .F. ) ;
#51950=FACE_OUTER_BOUND ( 'NONE', #80554, .T. ) ;
#52360=EDGE_CURVE ( 'NONE', #77270, #21926, #15626, .T. ) ;
#52392=CARTESIAN_POINT ( 'NONE',  ( 29.33919985515026596, -285.8906705383787994, 54.50000000000000711 ) ) ;
#52395=CYLINDRICAL_SURFACE ( 'NONE', #2043, 4.999999999999997335 ) ;
#52443=DIRECTION ( 'NONE',  ( -0.000000000000000000, -0.000000000000000000, -1.000000000000000000 ) ) ;
#52524=EDGE_CURVE ( 'NONE', #39706, #36049, #87572, .T. ) ;
#52548=LINE ( 'NONE', #45909, #64752 ) ;
#52624=EDGE_CURVE ( 'NONE', #84200, #36049, #51591, .T. ) ;
#52673=ORIENTED_EDGE ( 'NONE', *, *, #55414, .F. ) ;
#52696=VERTEX_POINT ( 'NONE', #45888 ) ;
#52714=FACE_OUTER_BOUND ( 'NONE', #6319, .T. ) ;
#53096=VECTOR ( 'NONE', #53842, 1000.000000000000000 ) ;
#53233=EDGE_CURVE ( 'NONE', #90307, #93354, #76647, .T. ) ;
#53315=CARTESIAN_POINT ( 'NONE',  ( -5.802570524182335987, -229.5268262511776527, 25.50000000000000000 ) ) ;
#53323=CARTESIAN_POINT ( 'NONE',  ( 11.63197158325052172, -331.8906705383788562, 52.50000000000000711 ) ) ;
#53333=CARTESIAN_POINT ( 'NONE',  ( -5.802570524182335987, -229.5268262511776527, 22.50000000000000000 ) ) ;
#53442=DIRECTION ( 'NONE',  ( -0.000000000000000000, 1.000000000000000000, -0.000000000000000000 ) ) ;
#53687=VECTOR ( 'NONE', #31628, 1000.000000000000000 ) ;
#53780=CARTESIAN_POINT ( 'NONE',  ( 29.33919985515026596, -285.8906705383787994, 27.50000000000000000 ) ) ;
#53842=DIRECTION ( 'NONE',  ( -0.000000000000000000, -0.000000000000000000, 1.000000000000000000 ) ) ;
#53971=SHAPE_DEFINITION_REPRESENTATION ( #12657, #71246 ) ;
#53976=CARTESIAN_POINT ( 'NONE',  ( 11.63197158325052172, -285.8906705383787994, 47.50000000000000711 ) ) ;
#54158=EDGE_LOOP ( 'NONE', ( #52673, #10083 ) ) ;
#54327=CARTESIAN_POINT ( 'NONE',  ( 11.63197158325052172, -282.8906705383787994, 47.50000000000000711 ) ) ;
#54387=VECTOR ( 'NONE', #81869, 1000.000000000000000 ) ;
#54403=ORIENTED_EDGE ( 'NONE', *, *, #49364, .T. ) ;
#54530=ORIENTED_EDGE ( 'NONE', *, *, #16849, .F. ) ;
#54549=DIRECTION ( 'NONE',  ( -0.000000000000000000, -1.000000000000000000, 0.000000000000000000 ) ) ;
#54820=DIRECTION ( 'NONE',  ( 0.000000000000000000, 0.000000000000000000, 1.000000000000000000 ) ) ;
#54853=ORIENTED_EDGE ( 'NONE', *, *, #3472, .T. ) ;
#54918=EDGE_LOOP ( 'NONE', ( #20772, #48747, #35899, #1578 ) ) ;
#54929=DIRECTION ( 'NONE',  ( -1.000000000000000000, 0.000000000000000000, 0.000000000000000000 ) ) ;
#54947=DIRECTION ( 'NONE',  ( 0.000000000000000000, 0.000000000000000000, 1.000000000000000000 ) ) ;
#55414=EDGE_CURVE ( 'NONE', #79053, #2187, #6157, .T. ) ;
#55446=EDGE_CURVE ( 'NONE', #34536, #33107, #84795, .T. ) ;
#55497=CARTESIAN_POINT ( 'NONE',  ( 9.339199855150265961, -212.1443419142231051, 22.50000000000000000 ) ) ;
#55521=ORIENTED_EDGE ( 'NONE', *, *, #21095, .T. ) ;
#55551=LINE ( 'NONE', #5370, #26154 ) ;
#55645=DIRECTION ( 'NONE',  ( -0.000000000000000000, 1.000000000000000000, -0.000000000000000000 ) ) ;
#55727=CARTESIAN_POINT ( 'NONE',  ( -74.94434090351494149, -212.1443419142231051, 54.50000000000000711 ) ) ;
#55983=CARTESIAN_POINT ( 'NONE',  ( -55.80257052418233599, -229.5268262511776527, 25.50000000000000000 ) ) ;
#56116=AXIS2_PLACEMENT_3D ( 'NONE', #63195, #5880, #92025 ) ;
#56119=DIRECTION ( 'NONE',  ( -0.000000000000000000, -0.000000000000000000, -1.000000000000000000 ) ) ;
#56443=AXIS2_PLACEMENT_3D ( 'NONE', #22241, #92919, #72895 ) ;
#56506=DIRECTION ( 'NONE',  ( 0.000000000000000000, 0.000000000000000000, -1.000000000000000000 ) ) ;
#56599=CARTESIAN_POINT ( 'NONE',  ( 11.63197158325052172, -331.8906705383788562, 47.50000000000000711 ) ) ;
#56813=EDGE_CURVE ( 'NONE', #9133, #2187, #48225, .T. ) ;
#56892=AXIS2_PLACEMENT_3D ( 'NONE', #24492, #90726, #25886 ) ;
#56976=CYLINDRICAL_SURFACE ( 'NONE', #42631, 8.000000000000000000 ) ;
#57245=DIRECTION ( 'NONE',  ( 1.000000000000000000, 0.000000000000000000, 0.000000000000000000 ) ) ;
#57377=( NAMED_UNIT ( * ) SI_UNIT ( $, .STERADIAN. ) SOLID_ANGLE_UNIT ( ) );
#57541=DIRECTION ( 'NONE',  ( 1.000000000000000000, 0.000000000000000000, 0.000000000000000000 ) ) ;
#57750=EDGE_CURVE ( 'NONE', #75426, #46169, #211, .T. ) ;
#57800=AXIS2_PLACEMENT_3D ( 'NONE', #88125, #594, #36561 ) ;
#57802=DIRECTION ( 'NONE',  ( 0.000000000000000000, 0.000000000000000000, 1.000000000000000000 ) ) ;
#57882=CARTESIAN_POINT ( 'NONE',  ( -74.94434090351494149, -282.8906705383787994, 30.50000000000000000 ) ) ;
#57977=EDGE_CURVE ( 'NONE', #8225, #45777, #83634, .T. ) ;
#58106=DIRECTION ( 'NONE',  ( -1.000000000000000000, -0.000000000000000000, -0.000000000000000000 ) ) ;
#58135=CARTESIAN_POINT ( 'NONE',  ( 9.339199855150265961, -282.8906705383787994, 54.50000000000000711 ) ) ;
#58223=CARTESIAN_POINT ( 'NONE',  ( -54.94434090351493438, -212.1443419142231051, 25.50000000000000000 ) ) ;
#58263=DIRECTION ( 'NONE',  ( -1.000000000000000000, 0.000000000000000000, -0.000000000000000000 ) ) ;
#58350=ORIENTED_EDGE ( 'NONE', *, *, #3216, .F. ) ;
#58435=VECTOR ( 'NONE', #18328, 1000.000000000000000 ) ;
#58445=ORIENTED_EDGE ( 'NONE', *, *, #35319, .T. ) ;
#58558=ADVANCED_FACE ( 'NONE', ( #35649 ), #56976, .F. ) ;
#58733=ADVANCED_FACE ( 'NONE', ( #79206 ), #35167, .T. ) ;
#58819=CARTESIAN_POINT ( 'NONE',  ( -54.94434090351493438, -212.1443419142231051, 25.50000000000000000 ) ) ;
#59068=ADVANCED_FACE ( 'NONE', ( #15723, #87204, #8145 ), #74394, .F. ) ;
#59082=VECTOR ( 'NONE', #34287, 1000.000000000000000 ) ;
#59378=LINE ( 'NONE', #1600, #47206 ) ;
#59496=EDGE_CURVE ( 'NONE', #39706, #83798, #62315, .T. ) ;
#60501=LINE ( 'NONE', #89817, #58435 ) ;
#60677=CARTESIAN_POINT ( 'NONE',  ( -54.94434090351493438, -282.8906705383787994, 54.50000000000000711 ) ) ;
#60683=CARTESIAN_POINT ( 'NONE',  ( -57.23711263161519724, -331.8906705383788562, 57.50000000000000711 ) ) ;
#60990=AXIS2_PLACEMENT_3D ( 'NONE', #85356, #91015, #84400 ) ;
#61102=PRODUCT_CONTEXT ( 'NONE', #20284, 'mechanical' ) ;
#61290=VERTEX_POINT ( 'NONE', #53333 ) ;
#61328=ORIENTED_EDGE ( 'NONE', *, *, #59496, .T. ) ;
#61391=EDGE_CURVE ( 'NONE', #63080, #39909, #80477, .T. ) ;
#61680=ORIENTED_EDGE ( 'NONE', *, *, #87037, .F. ) ;
#61923=DIRECTION ( 'NONE',  ( 0.000000000000000000, -1.000000000000000000, 0.000000000000000000 ) ) ;
#62047=CARTESIAN_POINT ( 'NONE',  ( 11.63197158325052172, -282.8906705383787994, 57.50000000000000000 ) ) ;
#62253=AXIS2_PLACEMENT_3D ( 'NONE', #17403, #24967, #89327 ) ;
#62315=CIRCLE ( 'NONE', #25996, 20.00000000000000355 ) ;
#63080=VERTEX_POINT ( 'NONE', #24768 ) ;
#63173=FACE_OUTER_BOUND ( 'NONE', #24169, .T. ) ;
#63195=CARTESIAN_POINT ( 'NONE',  ( 11.63197158325052172, -331.8906705383788562, 52.50000000000000711 ) ) ;
#63257=DIRECTION ( 'NONE',  ( 0.000000000000000000, -0.000000000000000000, -1.000000000000000000 ) ) ;
#63310=ORIENTED_EDGE ( 'NONE', *, *, #49364, .F. ) ;
#63665=CYLINDRICAL_SURFACE ( 'NONE', #56116, 4.999999999999997335 ) ;
#63722=DIRECTION ( 'NONE',  ( 1.000000000000000000, -0.000000000000000000, 0.000000000000000000 ) ) ;
#63802=VERTEX_POINT ( 'NONE', #55983 ) ;
#63972=CIRCLE ( 'NONE', #23097, 20.00000000000000000 ) ;
#63999=AXIS2_PLACEMENT_3D ( 'NONE', #45513, #82457, #67339 ) ;
#64019=ORIENTED_EDGE ( 'NONE', *, *, #55446, .F. ) ;
#64119=PRODUCT ( 'L sheet band', 'L sheet band', '', ( #61102 ) ) ;
#64380=EDGE_LOOP ( 'NONE', ( #47507, #90954, #89437, #34208, #41988, #82153 ) ) ;
#64479=( GEOMETRIC_REPRESENTATION_CONTEXT ( 3 ) GLOBAL_UNCERTAINTY_ASSIGNED_CONTEXT ( ( #11310 ) ) GLOBAL_UNIT_ASSIGNED_CONTEXT ( ( #27421, #44863, #87941 ) ) REPRESENTATION_CONTEXT ( 'NONE', 'WORKASPACE' ) );
#64752=VECTOR ( 'NONE', #74815, 1000.000000000000000 ) ;
#65339=DIRECTION ( 'NONE',  ( -0.000000000000000000, -0.000000000000000000, 1.000000000000000000 ) ) ;
#65408=EDGE_CURVE ( 'NONE', #36970, #49439, #22216, .T. ) ;
#65442=ORIENTED_EDGE ( 'NONE', *, *, #22580, .F. ) ;
#65453=CARTESIAN_POINT ( 'NONE',  ( 29.33919985515026596, -212.1443419142231051, 22.50000000000000000 ) ) ;
#66123=ORIENTED_EDGE ( 'NONE', *, *, #72960, .T. ) ;
#66165=FACE_OUTER_BOUND ( 'NONE', #19629, .T. ) ;
#66263=CARTESIAN_POINT ( 'NONE',  ( 29.33919985515026596, -212.1443419142231051, 25.50000000000000000 ) ) ;
#66581=CARTESIAN_POINT ( 'NONE',  ( -39.80257052418233599, -229.5268262511776527, 25.50000000000000000 ) ) ;
#66952=EDGE_CURVE ( 'NONE', #43263, #70876, #50515, .T. ) ;
#67039=VECTOR ( 'NONE', #65339, 1000.000000000000000 ) ;
#67339=DIRECTION ( 'NONE',  ( 0.000000000000000000, 0.000000000000000000, 1.000000000000000000 ) ) ;
#67418=CARTESIAN_POINT ( 'NONE',  ( -74.94434090351494149, -285.8906705383787994, 74.50000000000001421 ) ) ;
#67603=LINE ( 'NONE', #2731, #2451 ) ;
#67884=ADVANCED_BREP_SHAPE_REPRESENTATION ( '', ( #91539, #18940 ), #2252 ) ;
#68204=ADVANCED_FACE ( 'NONE', ( #36198 ), #34338, .F. ) ;
#68634=DIRECTION ( 'NONE',  ( 0.000000000000000000, 0.000000000000000000, 1.000000000000000000 ) ) ;
#68659=ORIENTED_EDGE ( 'NONE', *, *, #92271, .T. ) ;
#69013=ORIENTED_EDGE ( 'NONE', *, *, #70809, .T. ) ;
#69031=ADVANCED_FACE ( 'NONE', ( #52714 ), #73589, .T. ) ;
#69873=CARTESIAN_POINT ( 'NONE',  ( -74.94434090351494149, -280.8906705383787994, 27.50000000000000000 ) ) ;
#70116=DIRECTION ( 'NONE',  ( 1.000000000000000000, 0.000000000000000000, 0.000000000000000000 ) ) ;
#70282=CARTESIAN_POINT ( 'NONE',  ( -57.23711263161519724, -282.8906705383787994, 52.50000000000000711 ) ) ;
#70378=LINE ( 'NONE', #19228, #45243 ) ;
#70738=CARTESIAN_POINT ( 'NONE',  ( 11.63197158325052172, -282.8906705383787994, 52.50000000000000711 ) ) ;
#70809=EDGE_CURVE ( 'NONE', #90307, #49439, #9395, .T. ) ;
#70876=VERTEX_POINT ( 'NONE', #31207 ) ;
#70886=ORIENTED_EDGE ( 'NONE', *, *, #791, .T. ) ;
#70934=DIRECTION ( 'NONE',  ( 0.000000000000000000, 0.000000000000000000, 1.000000000000000000 ) ) ;
#71135=EDGE_CURVE ( 'NONE', #49439, #52696, #91196, .T. ) ;
#71246=SHAPE_REPRESENTATION ( 'L sheet band', ( #18940 ), #2252 ) ;
#71298=CARTESIAN_POINT ( 'NONE',  ( -55.80257052418233599, -229.5268262511776527, 22.50000000000000000 ) ) ;
#71405=FACE_BOUND ( 'NONE', #81663, .T. ) ;
#71407=DIRECTION ( 'NONE',  ( 0.000000000000000000, 1.000000000000000000, 0.000000000000000000 ) ) ;
#71531=AXIS2_PLACEMENT_3D ( 'NONE', #50785, #6304, #21433 ) ;
#71549=CARTESIAN_POINT ( 'NONE',  ( -74.94434090351494149, -212.1443419142231051, 25.50000000000000000 ) ) ;
#72077=ORIENTED_EDGE ( 'NONE', *, *, #92813, .T. ) ;
#72216=DIRECTION ( 'NONE',  ( 0.000000000000000000, 1.000000000000000000, 0.000000000000000000 ) ) ;
#72557=DIRECTION ( 'NONE',  ( 1.000000000000000000, 0.000000000000000000, 0.000000000000000000 ) ) ;
#72576=ORIENTED_EDGE ( 'NONE', *, *, #30839, .F. ) ;
#72809=CARTESIAN_POINT ( 'NONE',  ( 9.339199855150262408, -282.8906705383787994, 74.50000000000001421 ) ) ;
#72895=DIRECTION ( 'NONE',  ( 0.000000000000000000, 0.000000000000000000, 1.000000000000000000 ) ) ;
#72924=CARTESIAN_POINT ( 'NONE',  ( 29.33919985515026596, -277.8906705383787994, 25.50000000000000000 ) ) ;
#72960=EDGE_CURVE ( 'NONE', #61290, #21738, #530, .T. ) ;
#72981=ORIENTED_EDGE ( 'NONE', *, *, #29881, .T. ) ;
#72985=ADVANCED_FACE ( 'NONE', ( #85470 ), #93037, .F. ) ;
#73099=CIRCLE ( 'NONE', #33753, 8.000000000000000000 ) ;
#73392=CARTESIAN_POINT ( 'NONE',  ( 11.63197158325052172, -285.8906705383787994, 52.50000000000000711 ) ) ;
#73589=CYLINDRICAL_SURFACE ( 'NONE', #9712, 5.000000000000000888 ) ;
#73745=DIRECTION ( 'NONE',  ( -0.000000000000000000, 1.000000000000000000, -0.000000000000000000 ) ) ;
#74032=DIRECTION ( 'NONE',  ( 1.000000000000000000, 0.000000000000000000, 0.000000000000000000 ) ) ;
#74313=ADVANCED_FACE ( 'NONE', ( #47953 ), #32371, .F. ) ;
#74394=PLANE ( 'NONE',  #57800 ) ;
#74457=VERTEX_POINT ( 'NONE', #26667 ) ;
#74458=VECTOR ( 'NONE', #74032, 1000.000000000000000 ) ;
#74495=LINE ( 'NONE', #67418, #74458 ) ;
#74524=AXIS2_PLACEMENT_3D ( 'NONE', #17920, #54820, #84630 ) ;
#74747=AXIS2_PLACEMENT_3D ( 'NONE', #20606, #56119, #42829 ) ;
#74815=DIRECTION ( 'NONE',  ( 0.000000000000000000, 1.000000000000000000, 0.000000000000000000 ) ) ;
#74935=VERTEX_POINT ( 'NONE', #41790 ) ;
#75426=VERTEX_POINT ( 'NONE', #53976 ) ;
#76225=ORIENTED_EDGE ( 'NONE', *, *, #89855, .F. ) ;
#76243=ORIENTED_EDGE ( 'NONE', *, *, #7662, .F. ) ;
#76284=CARTESIAN_POINT ( 'NONE',  ( 29.33919985515026596, -212.1443419142231051, 54.50000000000000711 ) ) ;
#76329=ORIENTED_EDGE ( 'NONE', *, *, #93158, .T. ) ;
#76387=ADVANCED_FACE ( 'NONE', ( #78164 ), #6190, .T. ) ;
#76391=FACE_BOUND ( 'NONE', #54158, .T. ) ;
#76530=CIRCLE ( 'NONE', #56892, 5.000000000000004441 ) ;
#76647=LINE ( 'NONE', #4211, #12155 ) ;
#76716=ADVANCED_FACE ( 'NONE', ( #85712 ), #27491, .F. ) ;
#76791=ORIENTED_EDGE ( 'NONE', *, *, #50265, .T. ) ;
#76793=ORIENTED_EDGE ( 'NONE', *, *, #55446, .T. ) ;
#76941=PRODUCT_DEFINITION_CONTEXT ( 'detailed design', #929, 'design' ) ;
#77062=ORIENTED_EDGE ( 'NONE', *, *, #25784, .T. ) ;
#77112=EDGE_LOOP ( 'NONE', ( #10503, #77062 ) ) ;
#77127=CARTESIAN_POINT ( 'NONE',  ( -57.23711263161519724, -331.8906705383788562, 47.50000000000000000 ) ) ;
#77270=VERTEX_POINT ( 'NONE', #36228 ) ;
#77514=ORIENTED_EDGE ( 'NONE', *, *, #81207, .F. ) ;
#77580=VECTOR ( 'NONE', #37356, 1000.000000000000000 ) ;
#77668=AXIS2_PLACEMENT_3D ( 'NONE', #26785, #25368, #83119 ) ;
#78164=FACE_OUTER_BOUND ( 'NONE', #12388, .T. ) ;
#78459=ORIENTED_EDGE ( 'NONE', *, *, #70809, .F. ) ;
#78571=ORIENTED_EDGE ( 'NONE', *, *, #32103, .T. ) ;
#78625=DIRECTION ( 'NONE',  ( 0.000000000000000000, -1.000000000000000000, 0.000000000000000000 ) ) ;
#78642=DIRECTION ( 'NONE',  ( 1.000000000000000000, 0.000000000000000000, 0.000000000000000000 ) ) ;
#78821=LINE ( 'NONE', #30027, #85000 ) ;
#79010=VECTOR ( 'NONE', #55645, 1000.000000000000000 ) ;
#79015=PLANE ( 'NONE',  #35584 ) ;
#79053=VERTEX_POINT ( 'NONE', #85833 ) ;
#79096=CARTESIAN_POINT ( 'NONE',  ( -54.94434090351493438, 0.000000000000000000, 54.50000000000000711 ) ) ;
#79181=LINE ( 'NONE', #65453, #45958 ) ;
#79206=FACE_OUTER_BOUND ( 'NONE', #33367, .T. ) ;
#79292=ADVANCED_FACE ( 'NONE', ( #43228 ), #2470, .F. ) ;
#79384=VECTOR ( 'NONE', #20206, 1000.000000000000000 ) ;
#79413=CARTESIAN_POINT ( 'NONE',  ( -74.94434090351494149, -280.8906705383787994, 22.50000000000000000 ) ) ;
#79429=PRODUCT_DEFINITION ( 'UNKNOWN', '', #28085, #76941 ) ;
#79480=EDGE_LOOP ( 'NONE', ( #34055, #90355, #70886, #9965 ) ) ;
#79678=EDGE_LOOP ( 'NONE', ( #66123, #33006 ) ) ;
#79734=ORIENTED_EDGE ( 'NONE', *, *, #10105, .T. ) ;
#79767=DIRECTION ( 'NONE',  ( 0.000000000000000000, 0.000000000000000000, 1.000000000000000000 ) ) ;
#80151=VECTOR ( 'NONE', #16099, 1000.000000000000000 ) ;
#80210=CARTESIAN_POINT ( 'NONE',  ( 10.19742947581766401, -229.5268262511776527, 22.50000000000000000 ) ) ;
#80216=CARTESIAN_POINT ( 'NONE',  ( 29.33919985515026596, -280.8906705383787994, 27.50000000000000000 ) ) ;
#80378=ORIENTED_EDGE ( 'NONE', *, *, #39536, .T. ) ;
#80424=AXIS2_PLACEMENT_3D ( 'NONE', #13640, #86044, #70934 ) ;
#80477=CIRCLE ( 'NONE', #24517, 20.00000000000000355 ) ;
#80554=EDGE_LOOP ( 'NONE', ( #51241, #25792, #12648, #48682 ) ) ;
#80773=CIRCLE ( 'NONE', #89816, 8.000000000000000000 ) ;
#80833=AXIS2_PLACEMENT_3D ( 'NONE', #73392, #23178, #7577 ) ;
#80845=EDGE_CURVE ( 'NONE', #52696, #77270, #85727, .T. ) ;
#80972=CARTESIAN_POINT ( 'NONE',  ( 29.33919985515026596, -232.1443419142230766, 25.50000000000000000 ) ) ;
#81041=AXIS2_PLACEMENT_3D ( 'NONE', #22181, #52443, #30676 ) ;
#81207=EDGE_CURVE ( 'NONE', #5562, #83883, #73099, .T. ) ;
#81403=ORIENTED_EDGE ( 'NONE', *, *, #32103, .F. ) ;
#81433=VERTEX_POINT ( 'NONE', #503 ) ;
#81498=LINE ( 'NONE', #60683, #83575 ) ;
#81663=EDGE_LOOP ( 'NONE', ( #15815, #17251 ) ) ;
#81732=CARTESIAN_POINT ( 'NONE',  ( -74.94434090351494149, -212.1443419142231051, 25.50000000000000000 ) ) ;
#81869=DIRECTION ( 'NONE',  ( -1.000000000000000000, 0.000000000000000000, 0.000000000000000000 ) ) ;
#81914=CARTESIAN_POINT ( 'NONE',  ( -74.94434090351494149, -232.1443419142230766, 22.50000000000000000 ) ) ;
#82008=ORIENTED_EDGE ( 'NONE', *, *, #57977, .T. ) ;
#82022=EDGE_LOOP ( 'NONE', ( #33313, #2764, #58350, #45293 ) ) ;
#82153=ORIENTED_EDGE ( 'NONE', *, *, #66952, .T. ) ;
#82457=DIRECTION ( 'NONE',  ( -0.000000000000000000, 1.000000000000000000, -0.000000000000000000 ) ) ;
#82507=DIRECTION ( 'NONE',  ( 0.000000000000000000, 0.000000000000000000, 1.000000000000000000 ) ) ;
#82550=DIRECTION ( 'NONE',  ( 0.000000000000000000, 0.000000000000000000, -1.000000000000000000 ) ) ;
#82780=DIRECTION ( 'NONE',  ( -0.000000000000000000, -0.000000000000000000, -1.000000000000000000 ) ) ;
#82979=CIRCLE ( 'NONE', #42152, 8.000000000000000000 ) ;
#83119=DIRECTION ( 'NONE',  ( 0.000000000000000000, 0.000000000000000000, 1.000000000000000000 ) ) ;
#83276=ORIENTED_EDGE ( 'NONE', *, *, #89855, .T. ) ;
#83322=VERTEX_POINT ( 'NONE', #72809 ) ;
#83487=EDGE_LOOP ( 'NONE', ( #12164, #55521, #76793, #65442 ) ) ;
#83569=CARTESIAN_POINT ( 'NONE',  ( 29.33919985515026596, -212.1443419142231051, 25.50000000000000000 ) ) ;
#83575=VECTOR ( 'NONE', #39326, 1000.000000000000000 ) ;
#83634=LINE ( 'NONE', #18797, #53096 ) ;
#83798=VERTEX_POINT ( 'NONE', #23071 ) ;
#83824=ADVANCED_FACE ( 'NONE', ( #51950 ), #88404, .F. ) ;
#83883=VERTEX_POINT ( 'NONE', #30653 ) ;
#83926=DIRECTION ( 'NONE',  ( 0.000000000000000000, 0.000000000000000000, 1.000000000000000000 ) ) ;
#84118=DIRECTION ( 'NONE',  ( -0.000000000000000000, -0.000000000000000000, -1.000000000000000000 ) ) ;
#84122=ORIENTED_EDGE ( 'NONE', *, *, #50265, .F. ) ;
#84200=VERTEX_POINT ( 'NONE', #47642 ) ;
#84400=DIRECTION ( 'NONE',  ( 0.000000000000000000, -0.000000000000000000, -1.000000000000000000 ) ) ;
#84423=ORIENTED_EDGE ( 'NONE', *, *, #57977, .F. ) ;
#84486=ORIENTED_EDGE ( 'NONE', *, *, #59496, .F. ) ;
#84579=CARTESIAN_POINT ( 'NONE',  ( 29.33919985515026596, -282.8906705383787994, 54.50000000000000711 ) ) ;
#84630=DIRECTION ( 'NONE',  ( -1.000000000000000000, 0.000000000000000000, 0.000000000000000000 ) ) ;
#84642=LINE ( 'NONE', #10810, #22975 ) ;
#84683=CARTESIAN_POINT ( 'NONE',  ( -47.80257052418233599, -229.5268262511776527, 25.50000000000000000 ) ) ;
#84795=CIRCLE ( 'NONE', #28872, 4.999999999999997335 ) ;
#84848=DIRECTION ( 'NONE',  ( 1.000000000000000000, 0.000000000000000000, 0.000000000000000000 ) ) ;
#85000=VECTOR ( 'NONE', #28635, 1000.000000000000000 ) ;
#85084=VECTOR ( 'NONE', #61923, 1000.000000000000000 ) ;
#85123=DIRECTION ( 'NONE',  ( -0.000000000000000000, 1.000000000000000000, -0.000000000000000000 ) ) ;
#85220=FACE_OUTER_BOUND ( 'NONE', #82022, .T. ) ;
#85356=CARTESIAN_POINT ( 'NONE',  ( -74.94434090351494149, -282.8906705383787994, 74.50000000000001421 ) ) ;
#85364=DIRECTION ( 'NONE',  ( -1.000000000000000000, 0.000000000000000000, 0.000000000000000000 ) ) ;
#85390=AXIS2_PLACEMENT_3D ( 'NONE', #84683, #68634, #11330 ) ;
#85419=ORIENTED_EDGE ( 'NONE', *, *, #35340, .F. ) ;
#85447=UNCERTAINTY_MEASURE_WITH_UNIT (LENGTH_MEASURE( 1.000000000000000082E-05 ), #20907, 'distance_accuracy_value', 'NONE');
#85470=FACE_OUTER_BOUND ( 'NONE', #41722, .T. ) ;
#85493=DIRECTION ( 'NONE',  ( 0.000000000000000000, 1.000000000000000000, -0.000000000000000000 ) ) ;
#85530=LINE ( 'NONE', #55727, #79384 ) ;
#85626=ORIENTED_EDGE ( 'NONE', *, *, #66952, .F. ) ;
#85712=FACE_OUTER_BOUND ( 'NONE', #93247, .T. ) ;
#85727=LINE ( 'NONE', #71549, #3535 ) ;
#85833=CARTESIAN_POINT ( 'NONE',  ( -57.23711263161519724, -282.8906705383787994, 57.50000000000000711 ) ) ;
#86044=DIRECTION ( 'NONE',  ( 0.000000000000000000, 1.000000000000000000, -0.000000000000000000 ) ) ;
#86046=DIRECTION ( 'NONE',  ( 0.000000000000000000, 0.000000000000000000, -1.000000000000000000 ) ) ;
#86118=ORIENTED_EDGE ( 'NONE', *, *, #80845, .F. ) ;
#86171=DIRECTION ( 'NONE',  ( 0.000000000000000000, 0.000000000000000000, -1.000000000000000000 ) ) ;
#86218=SHAPE_REPRESENTATION_RELATIONSHIP ( 'NONE' , 'NONE' ,  #71246, #67884 ) ;
#86276=CARTESIAN_POINT ( 'NONE',  ( -47.80257052418233599, -229.5268262511776527, 22.50000000000000000 ) ) ;
#86506=DIRECTION ( 'NONE',  ( 0.000000000000000000, 0.000000000000000000, 1.000000000000000000 ) ) ;
#86593=ORIENTED_EDGE ( 'NONE', *, *, #52524, .F. ) ;
#86710=AXIS2_PLACEMENT_3D ( 'NONE', #34589, #54947, #70116 ) ;
#86779=AXIS2_PLACEMENT_3D ( 'NONE', #33001, #17868, #90275 ) ;
#86938=CARTESIAN_POINT ( 'NONE',  ( 9.339199855150265961, -212.1443419142231051, 25.50000000000000000 ) ) ;
#87037=EDGE_CURVE ( 'NONE', #31343, #63802, #11303, .T. ) ;
#87204=FACE_BOUND ( 'NONE', #12043, .T. ) ;
#87304=DIRECTION ( 'NONE',  ( 0.000000000000000000, 0.000000000000000000, 1.000000000000000000 ) ) ;
#87350=EDGE_CURVE ( 'NONE', #83883, #5562, #91446, .T. ) ;
#87426=DIRECTION ( 'NONE',  ( -0.000000000000000000, -0.000000000000000000, -1.000000000000000000 ) ) ;
#87572=LINE ( 'NONE', #38319, #42296 ) ;
#87621=ORIENTED_EDGE ( 'NONE', *, *, #10105, .F. ) ;
#87941=( NAMED_UNIT ( * ) SI_UNIT ( $, .STERADIAN. ) SOLID_ANGLE_UNIT ( ) );
#88032=ORIENTED_EDGE ( 'NONE', *, *, #21756, .T. ) ;
#88052=CARTESIAN_POINT ( 'NONE',  ( 11.63197158325052172, -285.8906705383787994, 57.50000000000000000 ) ) ;
#88125=CARTESIAN_POINT ( 'NONE',  ( 0.000000000000000000, 0.000000000000000000, 25.50000000000000000 ) ) ;
#88183=ORIENTED_EDGE ( 'NONE', *, *, #15154, .T. ) ;
#88356=ADVANCED_FACE ( 'NONE', ( #3291, #34063, #50118 ), #79015, .T. ) ;
#88376=CARTESIAN_POINT ( 'NONE',  ( -74.94434090351494149, -285.8906705383787994, 54.50000000000000711 ) ) ;
#88404=CYLINDRICAL_SURFACE ( 'NONE', #29302, 5.000000000000004441 ) ;
#89289=DIRECTION ( 'NONE',  ( -0.000000000000000000, 0.000000000000000000, -1.000000000000000000 ) ) ;
#89327=DIRECTION ( 'NONE',  ( 0.000000000000000000, 0.000000000000000000, 1.000000000000000000 ) ) ;
#89437=ORIENTED_EDGE ( 'NONE', *, *, #21756, .F. ) ;
#89712=AXIS2_PLACEMENT_3D ( 'NONE', #34352, #79767, #57541 ) ;
#89815=DIRECTION ( 'NONE',  ( -1.000000000000000000, 0.000000000000000000, 0.000000000000000000 ) ) ;
#89816=AXIS2_PLACEMENT_3D ( 'NONE', #35139, #83926, #84848 ) ;
#89817=CARTESIAN_POINT ( 'NONE',  ( -39.80257052418233599, -229.5268262511776527, 25.50000000000000000 ) ) ;
#89855=EDGE_CURVE ( 'NONE', #39909, #81433, #2748, .T. ) ;
#90275=DIRECTION ( 'NONE',  ( 0.000000000000000000, 0.000000000000000000, -1.000000000000000000 ) ) ;
#90307=VERTEX_POINT ( 'NONE', #86938 ) ;
#90355=ORIENTED_EDGE ( 'NONE', *, *, #87037, .T. ) ;
#90624=ORIENTED_EDGE ( 'NONE', *, *, #92813, .F. ) ;
#90726=DIRECTION ( 'NONE',  ( -1.000000000000000000, 0.000000000000000000, 0.000000000000000000 ) ) ;
#90741=ORIENTED_EDGE ( 'NONE', *, *, #25784, .F. ) ;
#90759=CARTESIAN_POINT ( 'NONE',  ( 9.339199855150265961, -232.1443419142230766, 25.50000000000000000 ) ) ;
#90908=LINE ( 'NONE', #76284, #39699 ) ;
#90954=ORIENTED_EDGE ( 'NONE', *, *, #3216, .T. ) ;
#90959=CARTESIAN_POINT ( 'NONE',  ( 0.000000000000000000, 0.000000000000000000, 0.000000000000000000 ) ) ;
#91015=DIRECTION ( 'NONE',  ( 0.000000000000000000, -1.000000000000000000, 0.000000000000000000 ) ) ;
#91055=DIRECTION ( 'NONE',  ( 0.000000000000000000, 0.000000000000000000, 1.000000000000000000 ) ) ;
#91094=ORIENTED_EDGE ( 'NONE', *, *, #61391, .T. ) ;
#91196=CIRCLE ( 'NONE', #74524, 20.00000000000000355 ) ;
#91446=CIRCLE ( 'NONE', #9810, 8.000000000000000000 ) ;
#91539=MANIFOLD_SOLID_BREP ( 'Fillet14', #41575 ) ;
#91752=CYLINDRICAL_SURFACE ( 'NONE', #3654, 20.00000000000000355 ) ;
#91771=EDGE_LOOP ( 'NONE', ( #90624, #35614, #26205, #91094, #83276, #26379 ) ) ;
#91791=ORIENTED_EDGE ( 'NONE', *, *, #22448, .T. ) ;
#91837=ADVANCED_FACE ( 'NONE', ( #15534 ), #29758, .F. ) ;
#91928=CARTESIAN_POINT ( 'NONE',  ( 10.19742947581766401, -229.5268262511776527, 25.50000000000000000 ) ) ;
#92025=DIRECTION ( 'NONE',  ( 0.000000000000000000, 0.000000000000000000, 1.000000000000000000 ) ) ;
#92036=EDGE_LOOP ( 'NONE', ( #81403, #61680 ) ) ;
#92174=AXIS2_PLACEMENT_3D ( 'NONE', #49044, #85493, #20640 ) ;
#92271=EDGE_CURVE ( 'NONE', #31343, #16501, #60501, .T. ) ;
#92436=FACE_BOUND ( 'NONE', #39753, .T. ) ;
#92445=DIRECTION ( 'NONE',  ( -0.000000000000000000, -0.000000000000000000, -1.000000000000000000 ) ) ;
#92502=EDGE_CURVE ( 'NONE', #21926, #84200, #76530, .T. ) ;
#92639=VECTOR ( 'NONE', #63722, 1000.000000000000000 ) ;
#92813=EDGE_CURVE ( 'NONE', #16098, #74457, #67603, .T. ) ;
#92884=VERTEX_POINT ( 'NONE', #84579 ) ;
#92919=DIRECTION ( 'NONE',  ( 0.000000000000000000, 1.000000000000000000, -0.000000000000000000 ) ) ;
#93037=PLANE ( 'NONE',  #6628 ) ;
#93158=EDGE_CURVE ( 'NONE', #39909, #39706, #85530, .T. ) ;
#93247=EDGE_LOOP ( 'NONE', ( #91791, #32426, #7944, #76791 ) ) ;
#93354=VERTEX_POINT ( 'NONE', #55497 ) ;
#93760=COLOUR_RGB('Off White',0.89,0.88,0.83);
#93761=FILL_AREA_STYLE_COLOUR('',#93760);
#93762=FILL_AREA_STYLE('',(#93761));
#93763=SURFACE_STYLE_FILL_AREA(#93762);
#93764=SURFACE_SIDE_STYLE('',(#93763));
#93765=SURFACE_STYLE_USAGE(.BOTH.,#93764);
#93766=PRESENTATION_STYLE_ASSIGNMENT((#93765));
ENDSEC;
END-ISO-10303-21;
